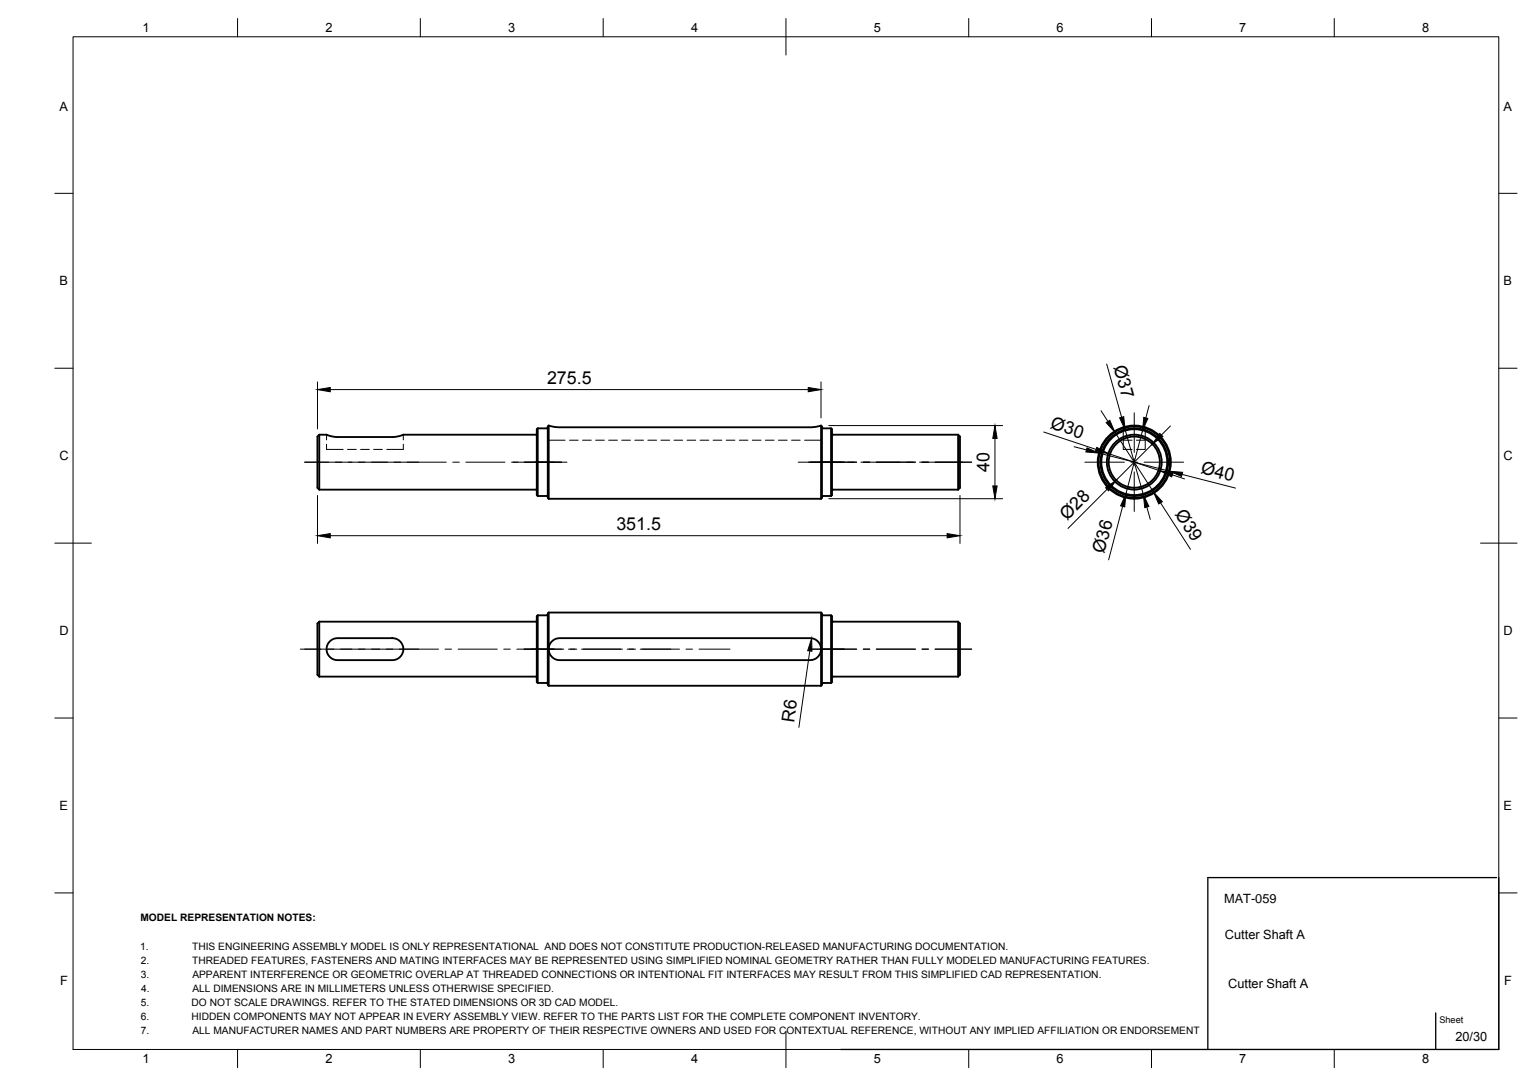
ISO-10303-21;
HEADER;
/* Generated by software containing ST-Developer
 * from STEP Tools, Inc. (www.steptools.com) 
 */

FILE_DESCRIPTION(
/* description */ ('', 'CAx-IF Rec.Pracs.---Representation and Presentation of Product Manufa
cturing Information (PMI)---4.0---2014-10-13'),
/* implementation_level */ '2;1');

FILE_NAME(
/* name */ 'Cutter Shaft A.step',
/* time_stamp */ '2026-10-28T23:00:48+01:00',
/* author */ (''),
/* organization */ (''),
/* preprocessor_version */ 'ST-DEVELOPER v20.2',
/* originating_system */ 'Autodesk Translation Framework v15.17.0.0',
/* authorisation */ '');

FILE_SCHEMA (('AP242_MANAGED_MODEL_BASED_3D_ENGINEERING_MIM_LF { 1 0 10303 442 2 1 4 }'));
ENDSEC;

DATA;
#10=MECHANICAL_DESIGN_GEOMETRIC_PRESENTATION_REPRESENTATION('',(#992),#61811);
#603=CONICAL_SURFACE('',#35992,18.25,0.785398163397426);
#604=CONICAL_SURFACE('',#35998,18.25,0.78539816339745);
#605=CONICAL_SURFACE('',#36004,14.5,0.785398163397442);
#606=CONICAL_SURFACE('',#36017,14.5,0.785398163397442);
#607=CONICAL_SURFACE('',#36025,19.75,0.78539816339745);
#608=CONICAL_SURFACE('',#36026,19.75,0.78539816339745);
#819=B_SPLINE_CURVE_WITH_KNOTS('',3,(#55896,#55897,#55898,#55899,#55900,
#55901,#55902,#55903,#55904,#55905),.UNSPECIFIED.,.F.,.F.,(4,2,2,2,4),(0.910129823137503,
1.1376283823127,1.36512694148791,1.59269329388146,1.82025964627501),
 .UNSPECIFIED.);
#820=B_SPLINE_CURVE_WITH_KNOTS('',3,(#55909,#55910,#55911,#55912,#55913,
#55914,#55915,#55916,#55917,#55918),.UNSPECIFIED.,.F.,.F.,(4,2,2,2,4),(1.82025964627501,
2.04782599866856,2.27539235106211,2.50289091023731,2.73038946941251),
 .UNSPECIFIED.);
#821=B_SPLINE_CURVE_WITH_KNOTS('',3,(#55923,#55924,#55925,#55926,#55927,
#55928,#55929,#55930,#55931,#55932,#55933,#55934,#55935,#55936,#55937,#55938,
#55939,#55940),.UNSPECIFIED.,.F.,.F.,(4,2,2,2,2,2,2,2,4),(0.,0.22893459915159,
0.45786919830318,0.68657220048275,0.91527520266232,1.14397820484189,1.37268120702146,
1.60161580617305,1.83055040532464),.UNSPECIFIED.);
#822=B_SPLINE_CURVE_WITH_KNOTS('',3,(#55959,#55960,#55961,#55962,#55963,
#55964,#55965,#55966,#55967,#55968,#55969,#55970,#55971,#55972,#55973,#55974,
#55975,#55976),.UNSPECIFIED.,.F.,.F.,(4,2,2,2,2,2,2,2,4),(-3.6611008106493,
-3.4321662114977,-3.20323161234611,-2.97452861016654,-2.74582560798697,
-2.5171226058074,-2.28841960362783,-2.05948500447624,-1.83055040532465),
 .UNSPECIFIED.);
#823=B_SPLINE_CURVE_WITH_KNOTS('',3,(#56047,#56048,#56049,#56050,#56051,
#56052,#56053,#56054,#56055,#56056),.UNSPECIFIED.,.F.,.F.,(4,2,2,2,4),(2.73038946941251,
2.95788802858771,3.18538658776291,3.41295294015646,3.64051929255001),
 .UNSPECIFIED.);
#824=B_SPLINE_CURVE_WITH_KNOTS('',3,(#56068,#56069,#56070,#56071,#56072,
#56073,#56074,#56075,#56076,#56077),.UNSPECIFIED.,.F.,.F.,(4,2,2,2,4),(0.,
0.22756635239355,0.4551327047871,0.682631263962301,0.910129823137503),
 .UNSPECIFIED.);
#898=TOROIDAL_SURFACE('',#35973,15.5,0.5);
#899=TOROIDAL_SURFACE('',#35982,15.5,0.5);
#900=TOROIDAL_SURFACE('',#36020,19.,0.500000000000029);
#901=TOROIDAL_SURFACE('',#36030,19.,0.499999999999998);
#928=SHAPE_REPRESENTATION_RELATIONSHIP('SRR','None',#61988,#953);
#953=ADVANCED_BREP_SHAPE_REPRESENTATION('',(#1031),#61801);
#992=STYLED_ITEM('',(#62156),#1031);
#1031=MANIFOLD_SOLID_BREP('Body1',#33822);
#1370=CYLINDRICAL_SURFACE('',#35963,20.);
#1371=CYLINDRICAL_SURFACE('',#35966,5.99999999999999);
#1372=CYLINDRICAL_SURFACE('',#35970,6.00000000000001);
#1373=CYLINDRICAL_SURFACE('',#35980,15.);
#1374=CYLINDRICAL_SURFACE('',#35989,15.);
#1375=CYLINDRICAL_SURFACE('',#35995,18.5);
#1376=CYLINDRICAL_SURFACE('',#36001,18.5);
#1377=CYLINDRICAL_SURFACE('',#36007,6.);
#1378=CYLINDRICAL_SURFACE('',#36011,6.);
#1379=CYLINDRICAL_SURFACE('',#36014,20.);
#2116=FACE_BOUND('',#7318,.T.);
#2117=FACE_BOUND('',#7320,.T.);
#2118=FACE_BOUND('',#7323,.T.);
#2119=FACE_BOUND('',#7341,.T.);
#2120=FACE_BOUND('',#7345,.T.);
#3038=CIRCLE('',#35964,20.);
#3039=CIRCLE('',#35965,20.);
#3040=CIRCLE('',#35967,5.99999999999999);
#3041=CIRCLE('',#35971,6.00000000000001);
#3042=CIRCLE('',#35974,15.);
#3043=CIRCLE('',#35975,15.);
#3044=CIRCLE('',#35976,0.5);
#3045=CIRCLE('',#35977,15.5);
#3046=CIRCLE('',#35979,18.);
#3047=CIRCLE('',#35981,15.);
#3048=CIRCLE('',#35983,15.5);
#3049=CIRCLE('',#35984,0.5);
#3050=CIRCLE('',#35985,15.);
#3051=CIRCLE('',#35986,15.);
#3052=CIRCLE('',#35988,18.);
#3053=CIRCLE('',#35990,15.);
#3054=CIRCLE('',#35991,15.);
#3055=CIRCLE('',#35993,18.5);
#3056=CIRCLE('',#35994,18.5);
#3057=CIRCLE('',#35996,18.5);
#3058=CIRCLE('',#35997,18.5);
#3059=CIRCLE('',#35999,18.5);
#3060=CIRCLE('',#36000,18.5);
#3061=CIRCLE('',#36002,18.5);
#3062=CIRCLE('',#36003,18.5);
#3063=CIRCLE('',#36005,14.);
#3064=CIRCLE('',#36008,6.);
#3065=CIRCLE('',#36012,6.);
#3066=CIRCLE('',#36015,20.);
#3067=CIRCLE('',#36016,20.);
#3068=CIRCLE('',#36018,14.);
#3069=CIRCLE('',#36021,19.);
#3070=CIRCLE('',#36022,0.500000000000029);
#3071=CIRCLE('',#36024,19.5);
#3072=CIRCLE('',#36027,19.5);
#3073=CIRCLE('',#36029,19.);
#3074=CIRCLE('',#36031,0.499999999999998);
#5194=FACE_OUTER_BOUND('',#7310,.T.);
#5195=FACE_OUTER_BOUND('',#7311,.T.);
#5196=FACE_OUTER_BOUND('',#7312,.T.);
#5197=FACE_OUTER_BOUND('',#7313,.T.);
#5198=FACE_OUTER_BOUND('',#7314,.T.);
#5199=FACE_OUTER_BOUND('',#7315,.T.);
#5200=FACE_OUTER_BOUND('',#7316,.T.);
#5201=FACE_OUTER_BOUND('',#7317,.T.);
#5202=FACE_OUTER_BOUND('',#7319,.T.);
#5203=FACE_OUTER_BOUND('',#7321,.T.);
#5204=FACE_OUTER_BOUND('',#7322,.T.);
#5205=FACE_OUTER_BOUND('',#7324,.T.);
#5206=FACE_OUTER_BOUND('',#7325,.T.);
#5207=FACE_OUTER_BOUND('',#7326,.T.);
#5208=FACE_OUTER_BOUND('',#7327,.T.);
#5209=FACE_OUTER_BOUND('',#7328,.T.);
#5210=FACE_OUTER_BOUND('',#7329,.T.);
#5211=FACE_OUTER_BOUND('',#7330,.T.);
#5212=FACE_OUTER_BOUND('',#7331,.T.);
#5213=FACE_OUTER_BOUND('',#7332,.T.);
#5214=FACE_OUTER_BOUND('',#7333,.T.);
#5215=FACE_OUTER_BOUND('',#7334,.T.);
#5216=FACE_OUTER_BOUND('',#7335,.T.);
#5217=FACE_OUTER_BOUND('',#7336,.T.);
#5218=FACE_OUTER_BOUND('',#7337,.T.);
#5219=FACE_OUTER_BOUND('',#7338,.T.);
#5220=FACE_OUTER_BOUND('',#7339,.T.);
#5221=FACE_OUTER_BOUND('',#7340,.T.);
#5222=FACE_OUTER_BOUND('',#7342,.T.);
#5223=FACE_OUTER_BOUND('',#7343,.T.);
#5224=FACE_OUTER_BOUND('',#7344,.T.);
#5225=FACE_OUTER_BOUND('',#7346,.T.);
#7310=EDGE_LOOP('',(#26242,#26243,#26244,#26245,#26246,#26247));
#7311=EDGE_LOOP('',(#26248,#26249,#26250,#26251));
#7312=EDGE_LOOP('',(#26252,#26253,#26254,#26255));
#7313=EDGE_LOOP('',(#26256,#26257,#26258,#26259));
#7314=EDGE_LOOP('',(#26260,#26261,#26262,#26263));
#7315=EDGE_LOOP('',(#26264,#26265,#26266,#26267));
#7316=EDGE_LOOP('',(#26268,#26269,#26270,#26271,#26272));
#7317=EDGE_LOOP('',(#26273));
#7318=EDGE_LOOP('',(#26274));
#7319=EDGE_LOOP('',(#26275,#26276,#26277,#26278,#26279));
#7320=EDGE_LOOP('',(#26280,#26281,#26282,#26283));
#7321=EDGE_LOOP('',(#26284,#26285,#26286,#26287,#26288));
#7322=EDGE_LOOP('',(#26289));
#7323=EDGE_LOOP('',(#26290));
#7324=EDGE_LOOP('',(#26291,#26292,#26293,#26294,#26295,#26296));
#7325=EDGE_LOOP('',(#26297,#26298,#26299,#26300,#26301));
#7326=EDGE_LOOP('',(#26302,#26303,#26304,#26305,#26306,#26307));
#7327=EDGE_LOOP('',(#26308,#26309,#26310,#26311,#26312));
#7328=EDGE_LOOP('',(#26313,#26314,#26315,#26316,#26317,#26318));
#7329=EDGE_LOOP('',(#26319,#26320,#26321,#26322,#26323));
#7330=EDGE_LOOP('',(#26324));
#7331=EDGE_LOOP('',(#26325,#26326,#26327,#26328,#26329));
#7332=EDGE_LOOP('',(#26330,#26331,#26332,#26333));
#7333=EDGE_LOOP('',(#26334,#26335,#26336,#26337));
#7334=EDGE_LOOP('',(#26338,#26339,#26340,#26341,#26342));
#7335=EDGE_LOOP('',(#26343,#26344,#26345,#26346));
#7336=EDGE_LOOP('',(#26347,#26348,#26349,#26350,#26351,#26352));
#7337=EDGE_LOOP('',(#26353,#26354,#26355,#26356));
#7338=EDGE_LOOP('',(#26357));
#7339=EDGE_LOOP('',(#26358,#26359,#26360,#26361,#26362));
#7340=EDGE_LOOP('',(#26363));
#7341=EDGE_LOOP('',(#26364));
#7342=EDGE_LOOP('',(#26365,#26366,#26367,#26368,#26369));
#7343=EDGE_LOOP('',(#26370,#26371,#26372,#26373,#26374));
#7344=EDGE_LOOP('',(#26375));
#7345=EDGE_LOOP('',(#26376));
#7346=EDGE_LOOP('',(#26377,#26378,#26379,#26380,#26381));
#9757=LINE('',#55892,#12304);
#9758=LINE('',#55907,#12305);
#9759=LINE('',#55942,#12306);
#9760=LINE('',#55945,#12307);
#9761=LINE('',#55948,#12308);
#9762=LINE('',#55950,#12309);
#9763=LINE('',#55951,#12310);
#9764=LINE('',#55954,#12311);
#9765=LINE('',#55956,#12312);
#9766=LINE('',#55957,#12313);
#9767=LINE('',#55993,#12314);
#9768=LINE('',#56007,#12315);
#9769=LINE('',#56016,#12316);
#9770=LINE('',#56021,#12317);
#9771=LINE('',#56028,#12318);
#9772=LINE('',#56031,#12319);
#9773=LINE('',#56037,#12320);
#9774=LINE('',#56042,#12321);
#9775=LINE('',#56046,#12322);
#9776=LINE('',#56059,#12323);
#9777=LINE('',#56061,#12324);
#9778=LINE('',#56062,#12325);
#9779=LINE('',#56065,#12326);
#9780=LINE('',#56066,#12327);
#9781=LINE('',#56085,#12328);
#9782=LINE('',#56096,#12329);
#9783=LINE('',#56099,#12330);
#12304=VECTOR('',#43281,20.);
#12305=VECTOR('',#43284,10.);
#12306=VECTOR('',#43289,10.);
#12307=VECTOR('',#43292,10.);
#12308=VECTOR('',#43295,10.);
#12309=VECTOR('',#43296,10.);
#12310=VECTOR('',#43297,10.);
#12311=VECTOR('',#43300,10.);
#12312=VECTOR('',#43301,10.);
#12313=VECTOR('',#43302,10.);
#12314=VECTOR('',#43327,15.);
#12315=VECTOR('',#43344,15.);
#12316=VECTOR('',#43355,18.25);
#12317=VECTOR('',#43360,18.5);
#12318=VECTOR('',#43369,18.25);
#12319=VECTOR('',#43372,18.5);
#12320=VECTOR('',#43379,14.5);
#12321=VECTOR('',#43386,10.);
#12322=VECTOR('',#43389,10.);
#12323=VECTOR('',#43392,10.);
#12324=VECTOR('',#43393,10.);
#12325=VECTOR('',#43394,10.);
#12326=VECTOR('',#43397,10.);
#12327=VECTOR('',#43398,10.);
#12328=VECTOR('',#43413,14.5);
#12329=VECTOR('',#43430,19.75);
#12330=VECTOR('',#43433,19.75);
#15002=VERTEX_POINT('',#55890);
#15003=VERTEX_POINT('',#55891);
#15004=VERTEX_POINT('',#55893);
#15005=VERTEX_POINT('',#55895);
#15006=VERTEX_POINT('',#55906);
#15007=VERTEX_POINT('',#55908);
#15008=VERTEX_POINT('',#55921);
#15009=VERTEX_POINT('',#55922);
#15010=VERTEX_POINT('',#55941);
#15011=VERTEX_POINT('',#55943);
#15012=VERTEX_POINT('',#55947);
#15013=VERTEX_POINT('',#55949);
#15014=VERTEX_POINT('',#55953);
#15015=VERTEX_POINT('',#55955);
#15016=VERTEX_POINT('',#55980);
#15017=VERTEX_POINT('',#55981);
#15018=VERTEX_POINT('',#55984);
#15019=VERTEX_POINT('',#55988);
#15020=VERTEX_POINT('',#55991);
#15021=VERTEX_POINT('',#55995);
#15022=VERTEX_POINT('',#55997);
#15023=VERTEX_POINT('',#55999);
#15024=VERTEX_POINT('',#56003);
#15025=VERTEX_POINT('',#56006);
#15026=VERTEX_POINT('',#56008);
#15027=VERTEX_POINT('',#56012);
#15028=VERTEX_POINT('',#56013);
#15029=VERTEX_POINT('',#56018);
#15030=VERTEX_POINT('',#56019);
#15031=VERTEX_POINT('',#56024);
#15032=VERTEX_POINT('',#56025);
#15033=VERTEX_POINT('',#56030);
#15034=VERTEX_POINT('',#56032);
#15035=VERTEX_POINT('',#56036);
#15036=VERTEX_POINT('',#56041);
#15037=VERTEX_POINT('',#56043);
#15038=VERTEX_POINT('',#56045);
#15039=VERTEX_POINT('',#56058);
#15040=VERTEX_POINT('',#56060);
#15041=VERTEX_POINT('',#56064);
#15042=VERTEX_POINT('',#56084);
#15043=VERTEX_POINT('',#56089);
#15044=VERTEX_POINT('',#56093);
#15045=VERTEX_POINT('',#56098);
#15046=VERTEX_POINT('',#56102);
#19023=EDGE_CURVE('',#15002,#15003,#9757,.T.);
#19024=EDGE_CURVE('',#15004,#15002,#3038,.T.);
#19025=EDGE_CURVE('',#15004,#15005,#819,.T.);
#19026=EDGE_CURVE('',#15005,#15006,#9758,.T.);
#19027=EDGE_CURVE('',#15006,#15007,#820,.T.);
#19028=EDGE_CURVE('',#15007,#15003,#3039,.T.);
#19029=EDGE_CURVE('',#15008,#15009,#821,.T.);
#19030=EDGE_CURVE('',#15008,#15010,#9759,.T.);
#19031=EDGE_CURVE('',#15010,#15011,#3040,.T.);
#19032=EDGE_CURVE('',#15009,#15011,#9760,.T.);
#19033=EDGE_CURVE('',#15009,#15012,#9761,.T.);
#19034=EDGE_CURVE('',#15011,#15013,#9762,.T.);
#19035=EDGE_CURVE('',#15012,#15013,#9763,.T.);
#19036=EDGE_CURVE('',#15014,#15008,#9764,.T.);
#19037=EDGE_CURVE('',#15014,#15015,#9765,.T.);
#19038=EDGE_CURVE('',#15015,#15010,#9766,.T.);
#19039=EDGE_CURVE('',#15012,#15014,#822,.F.);
#19040=EDGE_CURVE('',#15013,#15015,#3041,.T.);
#19041=EDGE_CURVE('',#15016,#15017,#3042,.T.);
#19042=EDGE_CURVE('',#15017,#15016,#3043,.T.);
#19043=EDGE_CURVE('',#15016,#15018,#3044,.T.);
#19044=EDGE_CURVE('',#15018,#15018,#3045,.T.);
#19045=EDGE_CURVE('',#15019,#15019,#3046,.T.);
#19046=EDGE_CURVE('',#15020,#15020,#3047,.T.);
#19047=EDGE_CURVE('',#15020,#15017,#9767,.T.);
#19048=EDGE_CURVE('',#15021,#15021,#3048,.T.);
#19049=EDGE_CURVE('',#15021,#15022,#3049,.T.);
#19050=EDGE_CURVE('',#15022,#15023,#3050,.T.);
#19051=EDGE_CURVE('',#15023,#15022,#3051,.T.);
#19052=EDGE_CURVE('',#15024,#15024,#3052,.T.);
#19053=EDGE_CURVE('',#15023,#15025,#9768,.T.);
#19054=EDGE_CURVE('',#15026,#15025,#3053,.T.);
#19055=EDGE_CURVE('',#15025,#15026,#3054,.T.);
#19056=EDGE_CURVE('',#15027,#15028,#3055,.T.);
#19057=EDGE_CURVE('',#15028,#15027,#3056,.T.);
#19058=EDGE_CURVE('',#15027,#15024,#9769,.T.);
#19059=EDGE_CURVE('',#15029,#15030,#3057,.T.);
#19060=EDGE_CURVE('',#15029,#15028,#9770,.T.);
#19061=EDGE_CURVE('',#15030,#15029,#3058,.T.);
#19062=EDGE_CURVE('',#15031,#15032,#3059,.T.);
#19063=EDGE_CURVE('',#15032,#15031,#3060,.T.);
#19064=EDGE_CURVE('',#15031,#15019,#9771,.T.);
#19065=EDGE_CURVE('',#15032,#15033,#9772,.T.);
#19066=EDGE_CURVE('',#15033,#15034,#3061,.T.);
#19067=EDGE_CURVE('',#15034,#15033,#3062,.T.);
#19068=EDGE_CURVE('',#15026,#15035,#9773,.T.);
#19069=EDGE_CURVE('',#15035,#15035,#3063,.T.);
#19070=EDGE_CURVE('',#15006,#15036,#9774,.T.);
#19071=EDGE_CURVE('',#15036,#15037,#3064,.T.);
#19072=EDGE_CURVE('',#15038,#15037,#9775,.T.);
#19073=EDGE_CURVE('',#15007,#15038,#823,.T.);
#19074=EDGE_CURVE('',#15038,#15039,#9776,.T.);
#19075=EDGE_CURVE('',#15037,#15040,#9777,.T.);
#19076=EDGE_CURVE('',#15039,#15040,#9778,.T.);
#19077=EDGE_CURVE('',#15005,#15041,#9779,.T.);
#19078=EDGE_CURVE('',#15041,#15036,#9780,.T.);
#19079=EDGE_CURVE('',#15039,#15004,#824,.T.);
#19080=EDGE_CURVE('',#15040,#15041,#3065,.T.);
#19081=EDGE_CURVE('',#15003,#15007,#3066,.T.);
#19082=EDGE_CURVE('',#15002,#15004,#3067,.T.);
#19083=EDGE_CURVE('',#15020,#15042,#9781,.T.);
#19084=EDGE_CURVE('',#15042,#15042,#3068,.T.);
#19085=EDGE_CURVE('',#15043,#15043,#3069,.T.);
#19086=EDGE_CURVE('',#15043,#15030,#3070,.T.);
#19087=EDGE_CURVE('',#15044,#15044,#3071,.T.);
#19088=EDGE_CURVE('',#15003,#15044,#9782,.T.);
#19089=EDGE_CURVE('',#15002,#15045,#9783,.T.);
#19090=EDGE_CURVE('',#15045,#15045,#3072,.T.);
#19091=EDGE_CURVE('',#15046,#15046,#3073,.T.);
#19092=EDGE_CURVE('',#15034,#15046,#3074,.T.);
#26242=ORIENTED_EDGE('',*,*,#19023,.F.);
#26243=ORIENTED_EDGE('',*,*,#19024,.F.);
#26244=ORIENTED_EDGE('',*,*,#19025,.T.);
#26245=ORIENTED_EDGE('',*,*,#19026,.T.);
#26246=ORIENTED_EDGE('',*,*,#19027,.T.);
#26247=ORIENTED_EDGE('',*,*,#19028,.T.);
#26248=ORIENTED_EDGE('',*,*,#19029,.F.);
#26249=ORIENTED_EDGE('',*,*,#19030,.T.);
#26250=ORIENTED_EDGE('',*,*,#19031,.T.);
#26251=ORIENTED_EDGE('',*,*,#19032,.F.);
#26252=ORIENTED_EDGE('',*,*,#19033,.F.);
#26253=ORIENTED_EDGE('',*,*,#19032,.T.);
#26254=ORIENTED_EDGE('',*,*,#19034,.T.);
#26255=ORIENTED_EDGE('',*,*,#19035,.F.);
#26256=ORIENTED_EDGE('',*,*,#19036,.F.);
#26257=ORIENTED_EDGE('',*,*,#19037,.T.);
#26258=ORIENTED_EDGE('',*,*,#19038,.T.);
#26259=ORIENTED_EDGE('',*,*,#19030,.F.);
#26260=ORIENTED_EDGE('',*,*,#19039,.F.);
#26261=ORIENTED_EDGE('',*,*,#19035,.T.);
#26262=ORIENTED_EDGE('',*,*,#19040,.T.);
#26263=ORIENTED_EDGE('',*,*,#19037,.F.);
#26264=ORIENTED_EDGE('',*,*,#19034,.F.);
#26265=ORIENTED_EDGE('',*,*,#19031,.F.);
#26266=ORIENTED_EDGE('',*,*,#19038,.F.);
#26267=ORIENTED_EDGE('',*,*,#19040,.F.);
#26268=ORIENTED_EDGE('',*,*,#19041,.T.);
#26269=ORIENTED_EDGE('',*,*,#19042,.T.);
#26270=ORIENTED_EDGE('',*,*,#19043,.T.);
#26271=ORIENTED_EDGE('',*,*,#19044,.T.);
#26272=ORIENTED_EDGE('',*,*,#19043,.F.);
#26273=ORIENTED_EDGE('',*,*,#19045,.F.);
#26274=ORIENTED_EDGE('',*,*,#19044,.F.);
#26275=ORIENTED_EDGE('',*,*,#19046,.F.);
#26276=ORIENTED_EDGE('',*,*,#19047,.T.);
#26277=ORIENTED_EDGE('',*,*,#19041,.F.);
#26278=ORIENTED_EDGE('',*,*,#19042,.F.);
#26279=ORIENTED_EDGE('',*,*,#19047,.F.);
#26280=ORIENTED_EDGE('',*,*,#19039,.T.);
#26281=ORIENTED_EDGE('',*,*,#19036,.T.);
#26282=ORIENTED_EDGE('',*,*,#19029,.T.);
#26283=ORIENTED_EDGE('',*,*,#19033,.T.);
#26284=ORIENTED_EDGE('',*,*,#19048,.T.);
#26285=ORIENTED_EDGE('',*,*,#19049,.T.);
#26286=ORIENTED_EDGE('',*,*,#19050,.T.);
#26287=ORIENTED_EDGE('',*,*,#19051,.T.);
#26288=ORIENTED_EDGE('',*,*,#19049,.F.);
#26289=ORIENTED_EDGE('',*,*,#19052,.F.);
#26290=ORIENTED_EDGE('',*,*,#19048,.F.);
#26291=ORIENTED_EDGE('',*,*,#19051,.F.);
#26292=ORIENTED_EDGE('',*,*,#19053,.T.);
#26293=ORIENTED_EDGE('',*,*,#19054,.F.);
#26294=ORIENTED_EDGE('',*,*,#19055,.F.);
#26295=ORIENTED_EDGE('',*,*,#19053,.F.);
#26296=ORIENTED_EDGE('',*,*,#19050,.F.);
#26297=ORIENTED_EDGE('',*,*,#19056,.T.);
#26298=ORIENTED_EDGE('',*,*,#19057,.T.);
#26299=ORIENTED_EDGE('',*,*,#19058,.T.);
#26300=ORIENTED_EDGE('',*,*,#19052,.T.);
#26301=ORIENTED_EDGE('',*,*,#19058,.F.);
#26302=ORIENTED_EDGE('',*,*,#19059,.F.);
#26303=ORIENTED_EDGE('',*,*,#19060,.T.);
#26304=ORIENTED_EDGE('',*,*,#19056,.F.);
#26305=ORIENTED_EDGE('',*,*,#19057,.F.);
#26306=ORIENTED_EDGE('',*,*,#19060,.F.);
#26307=ORIENTED_EDGE('',*,*,#19061,.F.);
#26308=ORIENTED_EDGE('',*,*,#19062,.T.);
#26309=ORIENTED_EDGE('',*,*,#19063,.T.);
#26310=ORIENTED_EDGE('',*,*,#19064,.T.);
#26311=ORIENTED_EDGE('',*,*,#19045,.T.);
#26312=ORIENTED_EDGE('',*,*,#19064,.F.);
#26313=ORIENTED_EDGE('',*,*,#19062,.F.);
#26314=ORIENTED_EDGE('',*,*,#19063,.F.);
#26315=ORIENTED_EDGE('',*,*,#19065,.T.);
#26316=ORIENTED_EDGE('',*,*,#19066,.T.);
#26317=ORIENTED_EDGE('',*,*,#19067,.T.);
#26318=ORIENTED_EDGE('',*,*,#19065,.F.);
#26319=ORIENTED_EDGE('',*,*,#19054,.T.);
#26320=ORIENTED_EDGE('',*,*,#19055,.T.);
#26321=ORIENTED_EDGE('',*,*,#19068,.T.);
#26322=ORIENTED_EDGE('',*,*,#19069,.T.);
#26323=ORIENTED_EDGE('',*,*,#19068,.F.);
#26324=ORIENTED_EDGE('',*,*,#19069,.F.);
#26325=ORIENTED_EDGE('',*,*,#19027,.F.);
#26326=ORIENTED_EDGE('',*,*,#19070,.T.);
#26327=ORIENTED_EDGE('',*,*,#19071,.T.);
#26328=ORIENTED_EDGE('',*,*,#19072,.F.);
#26329=ORIENTED_EDGE('',*,*,#19073,.F.);
#26330=ORIENTED_EDGE('',*,*,#19074,.F.);
#26331=ORIENTED_EDGE('',*,*,#19072,.T.);
#26332=ORIENTED_EDGE('',*,*,#19075,.T.);
#26333=ORIENTED_EDGE('',*,*,#19076,.F.);
#26334=ORIENTED_EDGE('',*,*,#19026,.F.);
#26335=ORIENTED_EDGE('',*,*,#19077,.T.);
#26336=ORIENTED_EDGE('',*,*,#19078,.T.);
#26337=ORIENTED_EDGE('',*,*,#19070,.F.);
#26338=ORIENTED_EDGE('',*,*,#19025,.F.);
#26339=ORIENTED_EDGE('',*,*,#19079,.F.);
#26340=ORIENTED_EDGE('',*,*,#19076,.T.);
#26341=ORIENTED_EDGE('',*,*,#19080,.T.);
#26342=ORIENTED_EDGE('',*,*,#19077,.F.);
#26343=ORIENTED_EDGE('',*,*,#19071,.F.);
#26344=ORIENTED_EDGE('',*,*,#19078,.F.);
#26345=ORIENTED_EDGE('',*,*,#19080,.F.);
#26346=ORIENTED_EDGE('',*,*,#19075,.F.);
#26347=ORIENTED_EDGE('',*,*,#19023,.T.);
#26348=ORIENTED_EDGE('',*,*,#19081,.T.);
#26349=ORIENTED_EDGE('',*,*,#19073,.T.);
#26350=ORIENTED_EDGE('',*,*,#19074,.T.);
#26351=ORIENTED_EDGE('',*,*,#19079,.T.);
#26352=ORIENTED_EDGE('',*,*,#19082,.F.);
#26353=ORIENTED_EDGE('',*,*,#19046,.T.);
#26354=ORIENTED_EDGE('',*,*,#19083,.T.);
#26355=ORIENTED_EDGE('',*,*,#19084,.F.);
#26356=ORIENTED_EDGE('',*,*,#19083,.F.);
#26357=ORIENTED_EDGE('',*,*,#19084,.T.);
#26358=ORIENTED_EDGE('',*,*,#19085,.F.);
#26359=ORIENTED_EDGE('',*,*,#19086,.T.);
#26360=ORIENTED_EDGE('',*,*,#19061,.T.);
#26361=ORIENTED_EDGE('',*,*,#19059,.T.);
#26362=ORIENTED_EDGE('',*,*,#19086,.F.);
#26363=ORIENTED_EDGE('',*,*,#19087,.F.);
#26364=ORIENTED_EDGE('',*,*,#19085,.T.);
#26365=ORIENTED_EDGE('',*,*,#19028,.F.);
#26366=ORIENTED_EDGE('',*,*,#19081,.F.);
#26367=ORIENTED_EDGE('',*,*,#19088,.T.);
#26368=ORIENTED_EDGE('',*,*,#19087,.T.);
#26369=ORIENTED_EDGE('',*,*,#19088,.F.);
#26370=ORIENTED_EDGE('',*,*,#19024,.T.);
#26371=ORIENTED_EDGE('',*,*,#19089,.T.);
#26372=ORIENTED_EDGE('',*,*,#19090,.F.);
#26373=ORIENTED_EDGE('',*,*,#19089,.F.);
#26374=ORIENTED_EDGE('',*,*,#19082,.T.);
#26375=ORIENTED_EDGE('',*,*,#19090,.T.);
#26376=ORIENTED_EDGE('',*,*,#19091,.F.);
#26377=ORIENTED_EDGE('',*,*,#19066,.F.);
#26378=ORIENTED_EDGE('',*,*,#19067,.F.);
#26379=ORIENTED_EDGE('',*,*,#19092,.T.);
#26380=ORIENTED_EDGE('',*,*,#19091,.T.);
#26381=ORIENTED_EDGE('',*,*,#19092,.F.);
#31625=PLANE('',#35968);
#31626=PLANE('',#35969);
#31627=PLANE('',#35972);
#31628=PLANE('',#35978);
#31629=PLANE('',#35987);
#31630=PLANE('',#36006);
#31631=PLANE('',#36009);
#31632=PLANE('',#36010);
#31633=PLANE('',#36013);
#31634=PLANE('',#36019);
#31635=PLANE('',#36023);
#31636=PLANE('',#36028);
#32875=ADVANCED_FACE('',(#5194),#1370,.T.);
#32876=ADVANCED_FACE('',(#5195),#1371,.F.);
#32877=ADVANCED_FACE('',(#5196),#31625,.F.);
#32878=ADVANCED_FACE('',(#5197),#31626,.F.);
#32879=ADVANCED_FACE('',(#5198),#1372,.F.);
#32880=ADVANCED_FACE('',(#5199),#31627,.F.);
#32881=ADVANCED_FACE('',(#5200),#898,.F.);
#32882=ADVANCED_FACE('',(#5201,#2116),#31628,.T.);
#32883=ADVANCED_FACE('',(#5202,#2117),#1373,.T.);
#32884=ADVANCED_FACE('',(#5203),#899,.F.);
#32885=ADVANCED_FACE('',(#5204,#2118),#31629,.T.);
#32886=ADVANCED_FACE('',(#5205),#1374,.T.);
#32887=ADVANCED_FACE('',(#5206),#603,.T.);
#32888=ADVANCED_FACE('',(#5207),#1375,.T.);
#32889=ADVANCED_FACE('',(#5208),#604,.T.);
#32890=ADVANCED_FACE('',(#5209),#1376,.T.);
#32891=ADVANCED_FACE('',(#5210),#605,.T.);
#32892=ADVANCED_FACE('',(#5211),#31630,.T.);
#32893=ADVANCED_FACE('',(#5212),#1377,.F.);
#32894=ADVANCED_FACE('',(#5213),#31631,.F.);
#32895=ADVANCED_FACE('',(#5214),#31632,.F.);
#32896=ADVANCED_FACE('',(#5215),#1378,.F.);
#32897=ADVANCED_FACE('',(#5216),#31633,.T.);
#32898=ADVANCED_FACE('',(#5217),#1379,.T.);
#32899=ADVANCED_FACE('',(#5218),#606,.T.);
#32900=ADVANCED_FACE('',(#5219),#31634,.T.);
#32901=ADVANCED_FACE('',(#5220),#900,.F.);
#32902=ADVANCED_FACE('',(#5221,#2119),#31635,.T.);
#32903=ADVANCED_FACE('',(#5222),#607,.T.);
#32904=ADVANCED_FACE('',(#5223),#608,.T.);
#32905=ADVANCED_FACE('',(#5224,#2120),#31636,.T.);
#32906=ADVANCED_FACE('',(#5225),#901,.F.);
#33822=CLOSED_SHELL('',(#32875,#32876,#32877,#32878,#32879,#32880,#32881,
#32882,#32883,#32884,#32885,#32886,#32887,#32888,#32889,#32890,#32891,#32892,
#32893,#32894,#32895,#32896,#32897,#32898,#32899,#32900,#32901,#32902,#32903,
#32904,#32905,#32906));
#35962=AXIS2_PLACEMENT_3D('',#55888,#43277,#43278);
#35963=AXIS2_PLACEMENT_3D('',#55889,#43279,#43280);
#35964=AXIS2_PLACEMENT_3D('',#55894,#43282,#43283);
#35965=AXIS2_PLACEMENT_3D('',#55919,#43285,#43286);
#35966=AXIS2_PLACEMENT_3D('',#55920,#43287,#43288);
#35967=AXIS2_PLACEMENT_3D('',#55944,#43290,#43291);
#35968=AXIS2_PLACEMENT_3D('',#55946,#43293,#43294);
#35969=AXIS2_PLACEMENT_3D('',#55952,#43298,#43299);
#35970=AXIS2_PLACEMENT_3D('',#55958,#43303,#43304);
#35971=AXIS2_PLACEMENT_3D('',#55977,#43305,#43306);
#35972=AXIS2_PLACEMENT_3D('',#55978,#43307,#43308);
#35973=AXIS2_PLACEMENT_3D('',#55979,#43309,#43310);
#35974=AXIS2_PLACEMENT_3D('',#55982,#43311,#43312);
#35975=AXIS2_PLACEMENT_3D('',#55983,#43313,#43314);
#35976=AXIS2_PLACEMENT_3D('',#55985,#43315,#43316);
#35977=AXIS2_PLACEMENT_3D('',#55986,#43317,#43318);
#35978=AXIS2_PLACEMENT_3D('',#55987,#43319,#43320);
#35979=AXIS2_PLACEMENT_3D('',#55989,#43321,#43322);
#35980=AXIS2_PLACEMENT_3D('',#55990,#43323,#43324);
#35981=AXIS2_PLACEMENT_3D('',#55992,#43325,#43326);
#35982=AXIS2_PLACEMENT_3D('',#55994,#43328,#43329);
#35983=AXIS2_PLACEMENT_3D('',#55996,#43330,#43331);
#35984=AXIS2_PLACEMENT_3D('',#55998,#43332,#43333);
#35985=AXIS2_PLACEMENT_3D('',#56000,#43334,#43335);
#35986=AXIS2_PLACEMENT_3D('',#56001,#43336,#43337);
#35987=AXIS2_PLACEMENT_3D('',#56002,#43338,#43339);
#35988=AXIS2_PLACEMENT_3D('',#56004,#43340,#43341);
#35989=AXIS2_PLACEMENT_3D('',#56005,#43342,#43343);
#35990=AXIS2_PLACEMENT_3D('',#56009,#43345,#43346);
#35991=AXIS2_PLACEMENT_3D('',#56010,#43347,#43348);
#35992=AXIS2_PLACEMENT_3D('',#56011,#43349,#43350);
#35993=AXIS2_PLACEMENT_3D('',#56014,#43351,#43352);
#35994=AXIS2_PLACEMENT_3D('',#56015,#43353,#43354);
#35995=AXIS2_PLACEMENT_3D('',#56017,#43356,#43357);
#35996=AXIS2_PLACEMENT_3D('',#56020,#43358,#43359);
#35997=AXIS2_PLACEMENT_3D('',#56022,#43361,#43362);
#35998=AXIS2_PLACEMENT_3D('',#56023,#43363,#43364);
#35999=AXIS2_PLACEMENT_3D('',#56026,#43365,#43366);
#36000=AXIS2_PLACEMENT_3D('',#56027,#43367,#43368);
#36001=AXIS2_PLACEMENT_3D('',#56029,#43370,#43371);
#36002=AXIS2_PLACEMENT_3D('',#56033,#43373,#43374);
#36003=AXIS2_PLACEMENT_3D('',#56034,#43375,#43376);
#36004=AXIS2_PLACEMENT_3D('',#56035,#43377,#43378);
#36005=AXIS2_PLACEMENT_3D('',#56038,#43380,#43381);
#36006=AXIS2_PLACEMENT_3D('',#56039,#43382,#43383);
#36007=AXIS2_PLACEMENT_3D('',#56040,#43384,#43385);
#36008=AXIS2_PLACEMENT_3D('',#56044,#43387,#43388);
#36009=AXIS2_PLACEMENT_3D('',#56057,#43390,#43391);
#36010=AXIS2_PLACEMENT_3D('',#56063,#43395,#43396);
#36011=AXIS2_PLACEMENT_3D('',#56067,#43399,#43400);
#36012=AXIS2_PLACEMENT_3D('',#56078,#43401,#43402);
#36013=AXIS2_PLACEMENT_3D('',#56079,#43403,#43404);
#36014=AXIS2_PLACEMENT_3D('',#56080,#43405,#43406);
#36015=AXIS2_PLACEMENT_3D('',#56081,#43407,#43408);
#36016=AXIS2_PLACEMENT_3D('',#56082,#43409,#43410);
#36017=AXIS2_PLACEMENT_3D('',#56083,#43411,#43412);
#36018=AXIS2_PLACEMENT_3D('',#56086,#43414,#43415);
#36019=AXIS2_PLACEMENT_3D('',#56087,#43416,#43417);
#36020=AXIS2_PLACEMENT_3D('',#56088,#43418,#43419);
#36021=AXIS2_PLACEMENT_3D('',#56090,#43420,#43421);
#36022=AXIS2_PLACEMENT_3D('',#56091,#43422,#43423);
#36023=AXIS2_PLACEMENT_3D('',#56092,#43424,#43425);
#36024=AXIS2_PLACEMENT_3D('',#56094,#43426,#43427);
#36025=AXIS2_PLACEMENT_3D('',#56095,#43428,#43429);
#36026=AXIS2_PLACEMENT_3D('',#56097,#43431,#43432);
#36027=AXIS2_PLACEMENT_3D('',#56100,#43434,#43435);
#36028=AXIS2_PLACEMENT_3D('',#56101,#43436,#43437);
#36029=AXIS2_PLACEMENT_3D('',#56103,#43438,#43439);
#36030=AXIS2_PLACEMENT_3D('',#56104,#43440,#43441);
#36031=AXIS2_PLACEMENT_3D('',#56105,#43442,#43443);
#43277=DIRECTION('axis',(0.,0.,1.));
#43278=DIRECTION('refdir',(1.,0.,0.));
#43279=DIRECTION('center_axis',(4.88578146679885E-16,1.,-9.3381869947186E-16));
#43280=DIRECTION('ref_axis',(1.,-4.8857814667989E-16,-5.46077161851014E-15));
#43281=DIRECTION('',(-4.88578146679885E-16,-1.,9.3381869947186E-16));
#43282=DIRECTION('center_axis',(4.88578146679885E-16,1.,-9.3381869947186E-16));
#43283=DIRECTION('ref_axis',(5.46077161851014E-15,9.33818699471857E-16,
1.));
#43284=DIRECTION('',(-4.88578146679885E-16,-1.,9.3381869947186E-16));
#43285=DIRECTION('center_axis',(4.88578146679885E-16,1.,-9.3381869947186E-16));
#43286=DIRECTION('ref_axis',(5.46077161851014E-15,9.33818699471857E-16,
1.));
#43287=DIRECTION('center_axis',(-1.,4.8857814667989E-16,5.46077161851014E-15));
#43288=DIRECTION('ref_axis',(4.88578146679884E-16,1.,-1.0562833793866E-15));
#43289=DIRECTION('',(-1.,4.8857814667989E-16,5.46077161851014E-15));
#43290=DIRECTION('center_axis',(-1.,4.8857814667989E-16,5.46077161851014E-15));
#43291=DIRECTION('ref_axis',(-4.88578146679885E-16,-1.,9.3381869947186E-16));
#43292=DIRECTION('',(-1.,4.8857814667989E-16,5.46077161851014E-15));
#43293=DIRECTION('center_axis',(-5.46077161851014E-15,-1.34090047516775E-15,
-1.));
#43294=DIRECTION('ref_axis',(-4.88578146679883E-16,-1.,1.34090047516775E-15));
#43295=DIRECTION('',(-4.88578146679885E-16,-1.,9.3381869947186E-16));
#43296=DIRECTION('',(-4.88578146679883E-16,-1.,1.34090047516775E-15));
#43297=DIRECTION('',(-1.,4.8857814667989E-16,5.46077161851014E-15));
#43298=DIRECTION('center_axis',(5.46077161851014E-15,1.2668856068594E-15,
1.));
#43299=DIRECTION('ref_axis',(4.88578146679883E-16,1.,-1.26688560685941E-15));
#43300=DIRECTION('',(4.88578146679885E-16,1.,-9.3381869947186E-16));
#43301=DIRECTION('',(-1.,4.8857814667989E-16,5.46077161851014E-15));
#43302=DIRECTION('',(4.88578146679883E-16,1.,-1.26688560685941E-15));
#43303=DIRECTION('center_axis',(-1.,4.8857814667989E-16,5.46077161851014E-15));
#43304=DIRECTION('ref_axis',(-4.88578146679885E-16,-1.,9.3381869947186E-16));
#43305=DIRECTION('center_axis',(-1.,4.8857814667989E-16,5.46077161851014E-15));
#43306=DIRECTION('ref_axis',(-4.88578146679885E-16,-1.,9.3381869947186E-16));
#43307=DIRECTION('center_axis',(-1.,4.14563278371546E-16,5.46077161851014E-15));
#43308=DIRECTION('ref_axis',(5.46077161851014E-15,9.33818699471857E-16,
1.));
#43309=DIRECTION('center_axis',(4.88578146679885E-16,1.,-9.3381869947186E-16));
#43310=DIRECTION('ref_axis',(3.5527136788005E-15,8.88178419700125E-16,1.));
#43311=DIRECTION('center_axis',(-4.88578146679885E-16,-1.,9.3381869947186E-16));
#43312=DIRECTION('ref_axis',(-1.,4.8857814667989E-16,5.27707459863804E-15));
#43313=DIRECTION('center_axis',(-4.88578146679885E-16,-1.,9.3381869947186E-16));
#43314=DIRECTION('ref_axis',(-1.,4.8857814667989E-16,5.27707459863804E-15));
#43315=DIRECTION('center_axis',(1.,-4.88578146679891E-16,-6.66133814775093E-15));
#43316=DIRECTION('ref_axis',(-6.66133814775093E-15,-1.11022302462516E-15,
-1.));
#43317=DIRECTION('center_axis',(4.88578146679885E-16,1.,-9.3381869947186E-16));
#43318=DIRECTION('ref_axis',(-1.,4.8857814667989E-16,5.27707459863804E-15));
#43319=DIRECTION('center_axis',(4.88578146679885E-16,1.,-9.3381869947186E-16));
#43320=DIRECTION('ref_axis',(5.46077161851014E-15,9.33818699471857E-16,
1.));
#43321=DIRECTION('center_axis',(-4.88578146679885E-16,-1.,9.3381869947186E-16));
#43322=DIRECTION('ref_axis',(-1.,4.8857814667989E-16,5.46077161851014E-15));
#43323=DIRECTION('center_axis',(4.88578146679885E-16,1.,-9.3381869947186E-16));
#43324=DIRECTION('ref_axis',(1.,-4.8857814667989E-16,-5.46077161851014E-15));
#43325=DIRECTION('center_axis',(4.88578146679885E-16,1.,-9.3381869947186E-16));
#43326=DIRECTION('ref_axis',(5.46077161851014E-15,9.33818699471857E-16,
1.));
#43327=DIRECTION('',(-4.88578146679885E-16,-1.,9.3381869947186E-16));
#43328=DIRECTION('center_axis',(4.88578146679885E-16,1.,-9.3381869947186E-16));
#43329=DIRECTION('ref_axis',(3.5527136788005E-15,0.,1.));
#43330=DIRECTION('center_axis',(-4.88578146679885E-16,-1.,9.3381869947186E-16));
#43331=DIRECTION('ref_axis',(-1.,4.8857814667989E-16,5.27707459863804E-15));
#43332=DIRECTION('center_axis',(1.,-4.88578146679891E-16,-6.66133814775093E-15));
#43333=DIRECTION('ref_axis',(-6.66133814775093E-15,0.,-1.));
#43334=DIRECTION('center_axis',(4.88578146679885E-16,1.,-9.3381869947186E-16));
#43335=DIRECTION('ref_axis',(-1.,4.8857814667989E-16,5.27707459863804E-15));
#43336=DIRECTION('center_axis',(4.88578146679885E-16,1.,-9.3381869947186E-16));
#43337=DIRECTION('ref_axis',(-1.,4.8857814667989E-16,5.27707459863804E-15));
#43338=DIRECTION('center_axis',(-4.88578146679885E-16,-1.,9.3381869947186E-16));
#43339=DIRECTION('ref_axis',(-5.46077161851014E-15,-9.33818699471857E-16,
-1.));
#43340=DIRECTION('center_axis',(4.88578146679885E-16,1.,-9.3381869947186E-16));
#43341=DIRECTION('ref_axis',(-1.,4.8857814667989E-16,5.46077161851014E-15));
#43342=DIRECTION('center_axis',(4.88578146679885E-16,1.,-9.3381869947186E-16));
#43343=DIRECTION('ref_axis',(1.,-4.8857814667989E-16,-5.46077161851014E-15));
#43344=DIRECTION('',(-4.88578146679885E-16,-1.,9.3381869947186E-16));
#43345=DIRECTION('center_axis',(-4.88578146679885E-16,-1.,9.3381869947186E-16));
#43346=DIRECTION('ref_axis',(-1.,4.8857814667989E-16,5.46077161851014E-15));
#43347=DIRECTION('center_axis',(-4.88578146679885E-16,-1.,9.3381869947186E-16));
#43348=DIRECTION('ref_axis',(-1.,4.8857814667989E-16,5.46077161851014E-15));
#43349=DIRECTION('center_axis',(4.88578146679885E-16,1.,-9.3381869947186E-16));
#43350=DIRECTION('ref_axis',(-1.,4.8857814667989E-16,5.46077161851014E-15));
#43351=DIRECTION('center_axis',(-4.88578146679885E-16,-1.,9.3381869947186E-16));
#43352=DIRECTION('ref_axis',(-1.,4.8857814667989E-16,5.46077161851014E-15));
#43353=DIRECTION('center_axis',(-4.88578146679885E-16,-1.,9.3381869947186E-16));
#43354=DIRECTION('ref_axis',(-1.,4.8857814667989E-16,5.46077161851014E-15));
#43355=DIRECTION('',(-0.707106781186532,-0.707106781186563,4.60825378237839E-15));
#43356=DIRECTION('center_axis',(4.88578146679885E-16,1.,-9.3381869947186E-16));
#43357=DIRECTION('ref_axis',(1.,-4.8857814667989E-16,-5.46077161851014E-15));
#43358=DIRECTION('center_axis',(4.88578146679885E-16,1.,-9.3381869947186E-16));
#43359=DIRECTION('ref_axis',(5.46077161851014E-15,9.33818699471857E-16,
1.));
#43360=DIRECTION('',(-4.88578146679885E-16,-1.,9.3381869947186E-16));
#43361=DIRECTION('center_axis',(4.88578146679885E-16,1.,-9.3381869947186E-16));
#43362=DIRECTION('ref_axis',(5.46077161851014E-15,9.33818699471857E-16,
1.));
#43363=DIRECTION('center_axis',(-4.88578146679885E-16,-1.,9.3381869947186E-16));
#43364=DIRECTION('ref_axis',(-1.,4.8857814667989E-16,5.46077161851014E-15));
#43365=DIRECTION('center_axis',(4.88578146679885E-16,1.,-9.3381869947186E-16));
#43366=DIRECTION('ref_axis',(-1.,4.8857814667989E-16,5.46077161851014E-15));
#43367=DIRECTION('center_axis',(4.88578146679885E-16,1.,-9.3381869947186E-16));
#43368=DIRECTION('ref_axis',(-1.,4.8857814667989E-16,5.46077161851014E-15));
#43369=DIRECTION('',(-0.707106781186548,0.707106781186547,3.11444350154066E-15));
#43370=DIRECTION('center_axis',(4.88578146679885E-16,1.,-9.3381869947186E-16));
#43371=DIRECTION('ref_axis',(1.,-4.8857814667989E-16,-5.46077161851014E-15));
#43372=DIRECTION('',(-4.88578146679885E-16,-1.,9.3381869947186E-16));
#43373=DIRECTION('center_axis',(4.88578146679885E-16,1.,-9.3381869947186E-16));
#43374=DIRECTION('ref_axis',(5.46077161851014E-15,9.33818699471857E-16,
1.));
#43375=DIRECTION('center_axis',(4.88578146679885E-16,1.,-9.3381869947186E-16));
#43376=DIRECTION('ref_axis',(5.46077161851014E-15,9.33818699471857E-16,
1.));
#43377=DIRECTION('center_axis',(4.88578146679885E-16,1.,-9.3381869947186E-16));
#43378=DIRECTION('ref_axis',(-1.,4.8857814667989E-16,5.46077161851014E-15));
#43379=DIRECTION('',(-0.707106781186543,-0.707106781186552,4.60825378237844E-15));
#43380=DIRECTION('center_axis',(4.88578146679885E-16,1.,-9.3381869947186E-16));
#43381=DIRECTION('ref_axis',(-1.,4.8857814667989E-16,5.46077161851014E-15));
#43382=DIRECTION('center_axis',(-4.88578146679885E-16,-1.,9.3381869947186E-16));
#43383=DIRECTION('ref_axis',(-5.46077161851014E-15,-9.33818699471857E-16,
-1.));
#43384=DIRECTION('center_axis',(-1.,4.8857814667989E-16,5.46077161851014E-15));
#43385=DIRECTION('ref_axis',(5.46077161851014E-15,9.33818699471857E-16,
1.));
#43386=DIRECTION('',(-1.,4.8857814667989E-16,5.46077161851014E-15));
#43387=DIRECTION('center_axis',(-1.,4.8857814667989E-16,5.46077161851014E-15));
#43388=DIRECTION('ref_axis',(5.46077161851014E-15,9.33818699471857E-16,
1.));
#43389=DIRECTION('',(-1.,4.8857814667989E-16,5.46077161851014E-15));
#43390=DIRECTION('center_axis',(5.46077161851014E-15,9.33818699471857E-16,
1.));
#43391=DIRECTION('ref_axis',(4.88578146679885E-16,1.,-9.3381869947186E-16));
#43392=DIRECTION('',(4.88578146679885E-16,1.,-9.3381869947186E-16));
#43393=DIRECTION('',(4.88578146679885E-16,1.,-9.3381869947186E-16));
#43394=DIRECTION('',(-1.,4.8857814667989E-16,5.46077161851014E-15));
#43395=DIRECTION('center_axis',(-5.46077161851014E-15,-9.33818699471857E-16,
-1.));
#43396=DIRECTION('ref_axis',(-4.88578146679885E-16,-1.,9.3381869947186E-16));
#43397=DIRECTION('',(-1.,4.8857814667989E-16,5.46077161851014E-15));
#43398=DIRECTION('',(-4.88578146679885E-16,-1.,9.3381869947186E-16));
#43399=DIRECTION('center_axis',(-1.,4.8857814667989E-16,5.46077161851014E-15));
#43400=DIRECTION('ref_axis',(-5.46077161851014E-15,-9.33818699471857E-16,
-1.));
#43401=DIRECTION('center_axis',(-1.,4.8857814667989E-16,5.46077161851014E-15));
#43402=DIRECTION('ref_axis',(-5.46077161851014E-15,-9.33818699471857E-16,
-1.));
#43403=DIRECTION('center_axis',(1.,-4.8857814667989E-16,-5.46077161851014E-15));
#43404=DIRECTION('ref_axis',(-5.46077161851014E-15,-9.33818699471857E-16,
-1.));
#43405=DIRECTION('center_axis',(4.88578146679885E-16,1.,-9.3381869947186E-16));
#43406=DIRECTION('ref_axis',(1.,-4.8857814667989E-16,-5.46077161851014E-15));
#43407=DIRECTION('center_axis',(4.88578146679885E-16,1.,-9.3381869947186E-16));
#43408=DIRECTION('ref_axis',(5.46077161851014E-15,9.33818699471857E-16,
1.));
#43409=DIRECTION('center_axis',(4.88578146679885E-16,1.,-9.3381869947186E-16));
#43410=DIRECTION('ref_axis',(5.46077161851014E-15,9.33818699471857E-16,
1.));
#43411=DIRECTION('center_axis',(-4.88578146679885E-16,-1.,9.3381869947186E-16));
#43412=DIRECTION('ref_axis',(1.,-4.8857814667989E-16,-5.46077161851014E-15));
#43413=DIRECTION('',(0.707106781186543,0.707106781186552,-4.43506257113134E-15));
#43414=DIRECTION('center_axis',(4.88578146679885E-16,1.,-9.3381869947186E-16));
#43415=DIRECTION('ref_axis',(5.46077161851014E-15,9.33818699471857E-16,
1.));
#43416=DIRECTION('center_axis',(4.88578146679885E-16,1.,-9.3381869947186E-16));
#43417=DIRECTION('ref_axis',(5.46077161851014E-15,9.33818699471857E-16,
1.));
#43418=DIRECTION('center_axis',(4.88578146679885E-16,1.,-9.3381869947186E-16));
#43419=DIRECTION('ref_axis',(5.83009424213414E-15,1.45752356053353E-15,
1.));
#43420=DIRECTION('center_axis',(4.88578146679885E-16,1.,-9.3381869947186E-16));
#43421=DIRECTION('ref_axis',(5.46077161851014E-15,9.33818699471858E-16,
1.));
#43422=DIRECTION('center_axis',(1.,-4.8857814667989E-16,-5.46571335200076E-15));
#43423=DIRECTION('ref_axis',(-5.46571335200076E-15,-1.82190445066692E-15,
-1.));
#43424=DIRECTION('center_axis',(-4.88578146679885E-16,-1.,9.3381869947186E-16));
#43425=DIRECTION('ref_axis',(-5.46077161851014E-15,-9.33818699471857E-16,
-1.));
#43426=DIRECTION('center_axis',(4.88578146679885E-16,1.,-9.3381869947186E-16));
#43427=DIRECTION('ref_axis',(5.46077161851014E-15,9.33818699471857E-16,
1.));
#43428=DIRECTION('center_axis',(4.88578146679885E-16,1.,-9.3381869947186E-16));
#43429=DIRECTION('ref_axis',(1.,-4.8857814667989E-16,-5.46077161851014E-15));
#43430=DIRECTION('',(0.707106781186548,-0.707106781186547,-3.28763471278776E-15));
#43431=DIRECTION('center_axis',(-4.88578146679885E-16,-1.,9.3381869947186E-16));
#43432=DIRECTION('ref_axis',(1.,-4.8857814667989E-16,-5.46077161851014E-15));
#43433=DIRECTION('',(0.707106781186549,0.707106781186546,-4.43506257113137E-15));
#43434=DIRECTION('center_axis',(4.88578146679885E-16,1.,-9.3381869947186E-16));
#43435=DIRECTION('ref_axis',(5.46077161851014E-15,9.33818699471857E-16,
1.));
#43436=DIRECTION('center_axis',(4.88578146679885E-16,1.,-9.3381869947186E-16));
#43437=DIRECTION('ref_axis',(5.46077161851014E-15,9.33818699471857E-16,
1.));
#43438=DIRECTION('center_axis',(4.88578146679885E-16,1.,-9.3381869947186E-16));
#43439=DIRECTION('ref_axis',(5.46077161851014E-15,9.33818699471858E-16,
1.));
#43440=DIRECTION('center_axis',(4.88578146679885E-16,1.,-9.3381869947186E-16));
#43441=DIRECTION('ref_axis',(5.83009424213416E-15,7.28761780266769E-16,
1.));
#43442=DIRECTION('center_axis',(1.,-4.8857814667989E-16,-5.46571335200076E-15));
#43443=DIRECTION('ref_axis',(-5.46571335200076E-15,-9.10952225333461E-16,
-1.));
#55888=CARTESIAN_POINT('',(0.,0.,0.));
#55889=CARTESIAN_POINT('Origin',(263.115917770968,-180.47200726879,445.000000551893));
#55890=CARTESIAN_POINT('',(243.115917770968,-105.97200726879,445.000000551893));
#55891=CARTESIAN_POINT('',(243.115917770968,-254.97200726879,445.000000551893));
#55892=CARTESIAN_POINT('',(243.115917770968,-180.47200726879,445.000000551893));
#55893=CARTESIAN_POINT('',(283.115917770968,-105.97200726879,445.000000551893));
#55894=CARTESIAN_POINT('Origin',(263.115917770968,-105.97200726879,445.000000551893));
#55895=CARTESIAN_POINT('',(282.194701799307,-111.97200726879,439.000000551893));
#55896=CARTESIAN_POINT('Ctrl Pts',(283.115917770968,-105.97200726879,445.000000551893));
#55897=CARTESIAN_POINT('Ctrl Pts',(283.115917770968,-105.97200726879,444.241672021309));
#55898=CARTESIAN_POINT('Ctrl Pts',(283.068520438725,-106.124510775769,443.435925116929));
#55899=CARTESIAN_POINT('Ctrl Pts',(282.89734167077,-106.738309454724,441.958955713881));
#55900=CARTESIAN_POINT('Ctrl Pts',(282.775789023268,-107.199354583986,441.287371862459));
#55901=CARTESIAN_POINT('Ctrl Pts',(282.545652805548,-108.259536519781,440.227189926664));
#55902=CARTESIAN_POINT('Ctrl Pts',(282.421616893032,-108.931056193358,439.766267099578));
#55903=CARTESIAN_POINT('Ctrl Pts',(282.244676552118,-110.407792297934,439.152558719695));
#55904=CARTESIAN_POINT('Ctrl Pts',(282.194701799307,-111.213452760811,439.000000551893));
#55905=CARTESIAN_POINT('Ctrl Pts',(282.194701799307,-111.97200726879,439.000000551893));
#55906=CARTESIAN_POINT('',(282.194701799307,-248.97200726879,439.000000551893));
#55907=CARTESIAN_POINT('',(282.194701799307,-180.47200726879,439.000000551893));
#55908=CARTESIAN_POINT('',(283.115917770968,-254.97200726879,445.000000551893));
#55909=CARTESIAN_POINT('Ctrl Pts',(282.194701799307,-248.97200726879,439.000000551893));
#55910=CARTESIAN_POINT('Ctrl Pts',(282.194701799307,-249.730561776769,439.000000551893));
#55911=CARTESIAN_POINT('Ctrl Pts',(282.244676552118,-250.536222239646,439.152558719695));
#55912=CARTESIAN_POINT('Ctrl Pts',(282.421616893032,-252.012958344222,439.766267099578));
#55913=CARTESIAN_POINT('Ctrl Pts',(282.545652805548,-252.684478017799,440.227189926664));
#55914=CARTESIAN_POINT('Ctrl Pts',(282.775789023268,-253.744659953594,441.287371862459));
#55915=CARTESIAN_POINT('Ctrl Pts',(282.89734167077,-254.205705082856,441.958955713881));
#55916=CARTESIAN_POINT('Ctrl Pts',(283.068520438725,-254.819503761811,443.435925116929));
#55917=CARTESIAN_POINT('Ctrl Pts',(283.115917770968,-254.97200726879,444.241672021309));
#55918=CARTESIAN_POINT('Ctrl Pts',(283.115917770968,-254.97200726879,445.000000551893));
#55919=CARTESIAN_POINT('Origin',(263.115917770968,-254.97200726879,445.000000551893));
#55920=CARTESIAN_POINT('Origin',(278.115917770968,9.52799273120991,445.000000551893));
#55921=CARTESIAN_POINT('',(276.863644855836,9.52799273120991,451.000000551893));
#55922=CARTESIAN_POINT('',(276.863644855836,9.52799273120991,439.000000551893));
#55923=CARTESIAN_POINT('Ctrl Pts',(276.863644855836,9.52799273120992,451.000000551893));
#55924=CARTESIAN_POINT('Ctrl Pts',(276.863644855836,10.2911080617152,451.000000551893));
#55925=CARTESIAN_POINT('Ctrl Pts',(276.933905272325,11.0983145255455,450.845735154055));
#55926=CARTESIAN_POINT('Ctrl Pts',(277.178138317006,12.5735133048384,450.230998285314));
#55927=CARTESIAN_POINT('Ctrl Pts',(277.347642076354,13.2423907504513,449.77088390689));
#55928=CARTESIAN_POINT('Ctrl Pts',(277.659025023679,14.2983417003919,448.714932956949));
#55929=CARTESIAN_POINT('Ctrl Pts',(277.822400067743,14.7588613493959,448.045853243948));
#55930=CARTESIAN_POINT('Ctrl Pts',(278.05222803659,15.3739084341755,446.569865474975));
#55931=CARTESIAN_POINT('Ctrl Pts',(278.115917770968,15.5279927312099,445.762343892491));
#55932=CARTESIAN_POINT('Ctrl Pts',(278.115917770968,15.5279927312099,444.237657211294));
#55933=CARTESIAN_POINT('Ctrl Pts',(278.05222803659,15.3739084341755,443.430135628811));
#55934=CARTESIAN_POINT('Ctrl Pts',(277.822400067743,14.7588613493959,441.954147859838));
#55935=CARTESIAN_POINT('Ctrl Pts',(277.659025023679,14.2983417003919,441.285068146836));
#55936=CARTESIAN_POINT('Ctrl Pts',(277.347642076353,13.2423907504513,440.229117196896));
#55937=CARTESIAN_POINT('Ctrl Pts',(277.178138317006,12.5735133048384,439.769002818472));
#55938=CARTESIAN_POINT('Ctrl Pts',(276.933905272324,11.0983145255455,439.154265949731));
#55939=CARTESIAN_POINT('Ctrl Pts',(276.863644855836,10.2911080617152,439.000000551893));
#55940=CARTESIAN_POINT('Ctrl Pts',(276.863644855836,9.52799273120991,439.000000551893));
#55941=CARTESIAN_POINT('',(270.115917770968,9.52799273120991,451.000000551893));
#55942=CARTESIAN_POINT('',(278.115917770968,9.52799273120991,451.000000551893));
#55943=CARTESIAN_POINT('',(270.115917770968,9.52799273120991,439.000000551893));
#55944=CARTESIAN_POINT('Origin',(270.115917770968,9.52799273120991,445.000000551893));
#55945=CARTESIAN_POINT('',(278.115917770968,9.52799273120991,439.000000551893));
#55946=CARTESIAN_POINT('Origin',(278.115917770968,9.52799273120991,439.000000551893));
#55947=CARTESIAN_POINT('',(276.863644855836,-20.4720072687901,439.000000551893));
#55948=CARTESIAN_POINT('',(276.863644855836,-39.9720072687901,439.000000551893));
#55949=CARTESIAN_POINT('',(270.115917770968,-20.4720072687901,439.000000551893));
#55950=CARTESIAN_POINT('',(270.115917770968,-20.4720072687901,439.000000551893));
#55951=CARTESIAN_POINT('',(278.115917770968,-20.4720072687901,439.000000551893));
#55952=CARTESIAN_POINT('Origin',(278.115917770968,-20.4720072687901,451.000000551893));
#55953=CARTESIAN_POINT('',(276.863644855836,-20.4720072687901,451.000000551893));
#55954=CARTESIAN_POINT('',(276.863644855836,-39.9720072687901,451.000000551893));
#55955=CARTESIAN_POINT('',(270.115917770968,-20.4720072687901,451.000000551893));
#55956=CARTESIAN_POINT('',(278.115917770968,-20.4720072687901,451.000000551893));
#55957=CARTESIAN_POINT('',(270.115917770968,9.52799273120991,451.000000551893));
#55958=CARTESIAN_POINT('Origin',(278.115917770968,-20.4720072687901,445.000000551893));
#55959=CARTESIAN_POINT('Ctrl Pts',(276.863644855836,-20.4720072687901,451.000000551893));
#55960=CARTESIAN_POINT('Ctrl Pts',(276.863644855836,-21.2351225992954,451.000000551893));
#55961=CARTESIAN_POINT('Ctrl Pts',(276.933905272325,-22.0423290631257,450.845735154055));
#55962=CARTESIAN_POINT('Ctrl Pts',(277.178138317006,-23.5175278424185,450.230998285314));
#55963=CARTESIAN_POINT('Ctrl Pts',(277.347642076354,-24.1864052880315,449.77088390689));
#55964=CARTESIAN_POINT('Ctrl Pts',(277.659025023679,-25.2423562379721,448.71493295695));
#55965=CARTESIAN_POINT('Ctrl Pts',(277.822400067743,-25.702875886976,448.045853243948));
#55966=CARTESIAN_POINT('Ctrl Pts',(278.05222803659,-26.3179229717557,446.569865474975));
#55967=CARTESIAN_POINT('Ctrl Pts',(278.115917770968,-26.4720072687901,445.762343892492));
#55968=CARTESIAN_POINT('Ctrl Pts',(278.115917770968,-26.4720072687901,444.237657211294));
#55969=CARTESIAN_POINT('Ctrl Pts',(278.05222803659,-26.3179229717557,443.430135628811));
#55970=CARTESIAN_POINT('Ctrl Pts',(277.822400067743,-25.702875886976,441.954147859838));
#55971=CARTESIAN_POINT('Ctrl Pts',(277.659025023679,-25.2423562379721,441.285068146836));
#55972=CARTESIAN_POINT('Ctrl Pts',(277.347642076353,-24.1864052880315,440.229117196896));
#55973=CARTESIAN_POINT('Ctrl Pts',(277.178138317006,-23.5175278424185,439.769002818472));
#55974=CARTESIAN_POINT('Ctrl Pts',(276.933905272324,-22.0423290631256,439.154265949731));
#55975=CARTESIAN_POINT('Ctrl Pts',(276.863644855836,-21.2351225992954,439.000000551893));
#55976=CARTESIAN_POINT('Ctrl Pts',(276.863644855836,-20.4720072687901,439.000000551893));
#55977=CARTESIAN_POINT('Origin',(270.115917770968,-20.4720072687901,445.000000551893));
#55978=CARTESIAN_POINT('Origin',(270.115917770968,-5.47200726879009,445.000000551893));
#55979=CARTESIAN_POINT('Origin',(263.115917770968,-98.97200726879,445.000000551893));
#55980=CARTESIAN_POINT('',(263.115917770968,-98.97200726879,430.000000551893));
#55981=CARTESIAN_POINT('',(248.115917770968,-98.97200726879,445.000000551893));
#55982=CARTESIAN_POINT('Origin',(263.115917770968,-98.97200726879,445.000000551893));
#55983=CARTESIAN_POINT('Origin',(263.115917770968,-98.97200726879,445.000000551893));
#55984=CARTESIAN_POINT('',(263.115917770968,-99.47200726879,429.500000551893));
#55985=CARTESIAN_POINT('Origin',(263.115917770968,-98.97200726879,429.500000551893));
#55986=CARTESIAN_POINT('Origin',(263.115917770968,-99.47200726879,445.000000551893));
#55987=CARTESIAN_POINT('Origin',(278.115917770968,-99.47200726879,445.000000551893));
#55988=CARTESIAN_POINT('',(281.115917770968,-99.47200726879,445.000000551893));
#55989=CARTESIAN_POINT('Origin',(263.115917770968,-99.47200726879,445.000000551893));
#55990=CARTESIAN_POINT('Origin',(263.115917770968,-39.9720072687901,445.000000551893));
#55991=CARTESIAN_POINT('',(248.115917770968,19.52799273121,445.000000551893));
#55992=CARTESIAN_POINT('Origin',(263.115917770968,19.5279927312099,445.000000551893));
#55993=CARTESIAN_POINT('',(248.115917770968,-39.9720072687901,445.000000551893));
#55994=CARTESIAN_POINT('Origin',(263.115917770968,-261.47200726879,445.000000551893));
#55995=CARTESIAN_POINT('',(263.115917770968,-260.97200726879,429.500000551893));
#55996=CARTESIAN_POINT('Origin',(263.115917770968,-260.97200726879,445.000000551893));
#55997=CARTESIAN_POINT('',(263.115917770968,-261.47200726879,430.000000551893));
#55998=CARTESIAN_POINT('Origin',(263.115917770968,-261.47200726879,429.500000551893));
#55999=CARTESIAN_POINT('',(248.115917770968,-261.47200726879,445.000000551893));
#56000=CARTESIAN_POINT('Origin',(263.115917770968,-261.47200726879,445.000000551893));
#56001=CARTESIAN_POINT('Origin',(263.115917770968,-261.47200726879,445.000000551893));
#56002=CARTESIAN_POINT('Origin',(281.615917770968,-260.97200726879,445.000000551893));
#56003=CARTESIAN_POINT('',(281.115917770968,-260.97200726879,445.000000551893));
#56004=CARTESIAN_POINT('Origin',(263.115917770968,-260.97200726879,445.000000551893));
#56005=CARTESIAN_POINT('Origin',(263.115917770968,-295.97200726879,445.000000551893));
#56006=CARTESIAN_POINT('',(248.115917770968,-329.97200726879,445.000000551893));
#56007=CARTESIAN_POINT('',(248.115917770968,-295.97200726879,445.000000551893));
#56008=CARTESIAN_POINT('',(278.115917770968,-329.97200726879,445.000000551893));
#56009=CARTESIAN_POINT('Origin',(263.115917770968,-329.97200726879,445.000000551893));
#56010=CARTESIAN_POINT('Origin',(263.115917770968,-329.97200726879,445.000000551893));
#56011=CARTESIAN_POINT('Origin',(263.115917770968,-260.72200726879,445.000000551893));
#56012=CARTESIAN_POINT('',(281.615917770968,-260.47200726879,445.000000551893));
#56013=CARTESIAN_POINT('',(244.615917770968,-260.47200726879,445.000000551893));
#56014=CARTESIAN_POINT('Origin',(263.115917770968,-260.47200726879,445.000000551893));
#56015=CARTESIAN_POINT('Origin',(263.115917770968,-260.47200726879,445.000000551893));
#56016=CARTESIAN_POINT('',(281.365917770968,-260.72200726879,445.000000551893));
#56017=CARTESIAN_POINT('Origin',(263.115917770968,-258.47200726879,445.000000551893));
#56018=CARTESIAN_POINT('',(244.615917770968,-255.97200726879,445.000000551893));
#56019=CARTESIAN_POINT('',(263.115917770968,-255.97200726879,426.500000551893));
#56020=CARTESIAN_POINT('Origin',(263.115917770968,-255.97200726879,445.000000551893));
#56021=CARTESIAN_POINT('',(244.615917770968,-258.47200726879,445.000000551893));
#56022=CARTESIAN_POINT('Origin',(263.115917770968,-255.97200726879,445.000000551893));
#56023=CARTESIAN_POINT('Origin',(263.115917770968,-99.72200726879,445.000000551893));
#56024=CARTESIAN_POINT('',(281.615917770968,-99.97200726879,445.000000551893));
#56025=CARTESIAN_POINT('',(244.615917770968,-99.97200726879,445.000000551893));
#56026=CARTESIAN_POINT('Origin',(263.115917770968,-99.97200726879,445.000000551893));
#56027=CARTESIAN_POINT('Origin',(263.115917770968,-99.97200726879,445.000000551893));
#56028=CARTESIAN_POINT('',(281.365917770968,-99.72200726879,445.000000551893));
#56029=CARTESIAN_POINT('Origin',(263.115917770968,-102.22200726879,445.000000551893));
#56030=CARTESIAN_POINT('',(244.615917770968,-104.97200726879,445.000000551893));
#56031=CARTESIAN_POINT('',(244.615917770968,-102.22200726879,445.000000551893));
#56032=CARTESIAN_POINT('',(263.115917770968,-104.97200726879,426.500000551893));
#56033=CARTESIAN_POINT('Origin',(263.115917770968,-104.97200726879,445.000000551893));
#56034=CARTESIAN_POINT('Origin',(263.115917770968,-104.97200726879,445.000000551893));
#56035=CARTESIAN_POINT('Origin',(263.115917770968,-330.47200726879,445.000000551893));
#56036=CARTESIAN_POINT('',(277.115917770968,-330.97200726879,445.000000551893));
#56037=CARTESIAN_POINT('',(277.615917770968,-330.47200726879,445.000000551893));
#56038=CARTESIAN_POINT('Origin',(263.115917770968,-330.97200726879,445.000000551893));
#56039=CARTESIAN_POINT('Origin',(278.115917770968,-330.97200726879,445.000000551893));
#56040=CARTESIAN_POINT('Origin',(283.115917770968,-248.97200726879,445.000000551893));
#56041=CARTESIAN_POINT('',(275.115917770968,-248.97200726879,439.000000551893));
#56042=CARTESIAN_POINT('',(283.115917770968,-248.97200726879,439.000000551893));
#56043=CARTESIAN_POINT('',(275.115917770968,-248.97200726879,451.000000551893));
#56044=CARTESIAN_POINT('Origin',(275.115917770968,-248.97200726879,445.000000551893));
#56045=CARTESIAN_POINT('',(282.194701799307,-248.97200726879,451.000000551893));
#56046=CARTESIAN_POINT('',(283.115917770968,-248.97200726879,451.000000551893));
#56047=CARTESIAN_POINT('Ctrl Pts',(283.115917770968,-254.97200726879,445.000000551893));
#56048=CARTESIAN_POINT('Ctrl Pts',(283.115917770968,-254.97200726879,445.758329082477));
#56049=CARTESIAN_POINT('Ctrl Pts',(283.068520438725,-254.819503761811,446.564075986857));
#56050=CARTESIAN_POINT('Ctrl Pts',(282.89734167077,-254.205705082856,448.041045389906));
#56051=CARTESIAN_POINT('Ctrl Pts',(282.775789023268,-253.744659953594,448.712629241327));
#56052=CARTESIAN_POINT('Ctrl Pts',(282.545652805548,-252.684478017799,449.772811177122));
#56053=CARTESIAN_POINT('Ctrl Pts',(282.421616893032,-252.012958344222,450.233734004208));
#56054=CARTESIAN_POINT('Ctrl Pts',(282.244676552118,-250.536222239646,450.847442384092));
#56055=CARTESIAN_POINT('Ctrl Pts',(282.194701799307,-249.730561776768,451.000000551893));
#56056=CARTESIAN_POINT('Ctrl Pts',(282.194701799307,-248.97200726879,451.000000551893));
#56057=CARTESIAN_POINT('Origin',(283.115917770968,-248.97200726879,451.000000551893));
#56058=CARTESIAN_POINT('',(282.194701799307,-111.97200726879,451.000000551893));
#56059=CARTESIAN_POINT('',(282.194701799307,-180.47200726879,451.000000551893));
#56060=CARTESIAN_POINT('',(275.115917770968,-111.97200726879,451.000000551893));
#56061=CARTESIAN_POINT('',(275.115917770968,-111.97200726879,451.000000551893));
#56062=CARTESIAN_POINT('',(283.115917770968,-111.97200726879,451.000000551893));
#56063=CARTESIAN_POINT('Origin',(283.115917770968,-111.97200726879,439.000000551893));
#56064=CARTESIAN_POINT('',(275.115917770968,-111.97200726879,439.000000551893));
#56065=CARTESIAN_POINT('',(283.115917770968,-111.97200726879,439.000000551893));
#56066=CARTESIAN_POINT('',(275.115917770968,-248.97200726879,439.000000551893));
#56067=CARTESIAN_POINT('Origin',(283.115917770968,-111.97200726879,445.000000551893));
#56068=CARTESIAN_POINT('Ctrl Pts',(282.194701799307,-111.97200726879,451.000000551893));
#56069=CARTESIAN_POINT('Ctrl Pts',(282.194701799307,-111.213452760811,451.000000551893));
#56070=CARTESIAN_POINT('Ctrl Pts',(282.244676552118,-110.407792297934,450.847442384091));
#56071=CARTESIAN_POINT('Ctrl Pts',(282.421616893032,-108.931056193358,450.233734004208));
#56072=CARTESIAN_POINT('Ctrl Pts',(282.545652805548,-108.259536519781,449.772811177122));
#56073=CARTESIAN_POINT('Ctrl Pts',(282.775789023268,-107.199354583986,448.712629241327));
#56074=CARTESIAN_POINT('Ctrl Pts',(282.89734167077,-106.738309454724,448.041045389905));
#56075=CARTESIAN_POINT('Ctrl Pts',(283.068520438725,-106.124510775769,446.564075986857));
#56076=CARTESIAN_POINT('Ctrl Pts',(283.115917770968,-105.97200726879,445.758329082477));
#56077=CARTESIAN_POINT('Ctrl Pts',(283.115917770968,-105.97200726879,445.000000551893));
#56078=CARTESIAN_POINT('Origin',(275.115917770968,-111.97200726879,445.000000551893));
#56079=CARTESIAN_POINT('Origin',(275.115917770968,-180.47200726879,445.000000551893));
#56080=CARTESIAN_POINT('Origin',(263.115917770968,-180.47200726879,445.000000551893));
#56081=CARTESIAN_POINT('Origin',(263.115917770968,-254.97200726879,445.000000551893));
#56082=CARTESIAN_POINT('Origin',(263.115917770968,-105.97200726879,445.000000551893));
#56083=CARTESIAN_POINT('Origin',(263.115917770968,20.0279927312099,445.000000551893));
#56084=CARTESIAN_POINT('',(249.115917770968,20.52799273121,445.000000551893));
#56085=CARTESIAN_POINT('',(248.615917770968,20.0279927312099,445.000000551893));
#56086=CARTESIAN_POINT('Origin',(263.115917770968,20.5279927312099,445.000000551893));
#56087=CARTESIAN_POINT('Origin',(263.115917770968,20.5279927312099,445.000000551893));
#56088=CARTESIAN_POINT('Origin',(263.115917770968,-255.97200726879,445.000000551893));
#56089=CARTESIAN_POINT('',(263.115917770968,-255.47200726879,426.000000551893));
#56090=CARTESIAN_POINT('Origin',(263.115917770968,-255.47200726879,445.000000551893));
#56091=CARTESIAN_POINT('Origin',(263.115917770968,-255.97200726879,426.000000551893));
#56092=CARTESIAN_POINT('Origin',(282.615917770968,-255.47200726879,445.000000551893));
#56093=CARTESIAN_POINT('',(243.615917770968,-255.47200726879,445.000000551893));
#56094=CARTESIAN_POINT('Origin',(263.115917770968,-255.47200726879,445.000000551893));
#56095=CARTESIAN_POINT('Origin',(263.115917770968,-255.22200726879,445.000000551893));
#56096=CARTESIAN_POINT('',(243.365917770968,-255.22200726879,445.000000551893));
#56097=CARTESIAN_POINT('Origin',(263.115917770968,-105.72200726879,445.000000551893));
#56098=CARTESIAN_POINT('',(243.615917770968,-105.47200726879,445.000000551893));
#56099=CARTESIAN_POINT('',(243.365917770968,-105.72200726879,445.000000551893));
#56100=CARTESIAN_POINT('Origin',(263.115917770968,-105.47200726879,445.000000551893));
#56101=CARTESIAN_POINT('Origin',(282.115917770968,-105.47200726879,445.000000551893));
#56102=CARTESIAN_POINT('',(263.115917770968,-105.47200726879,426.000000551893));
#56103=CARTESIAN_POINT('Origin',(263.115917770968,-105.47200726879,445.000000551893));
#56104=CARTESIAN_POINT('Origin',(263.115917770968,-104.97200726879,445.000000551893));
#56105=CARTESIAN_POINT('Origin',(263.115917770968,-104.97200726879,426.000000551893));
#61770=UNCERTAINTY_MEASURE_WITH_UNIT(LENGTH_MEASURE(0.01),#61812,
'DISTANCE_ACCURACY_VALUE',
'Maximum model space distance between geometric entities at asserted c
onnectivities');
#61780=UNCERTAINTY_MEASURE_WITH_UNIT(LENGTH_MEASURE(0.01),#61812,
'DISTANCE_ACCURACY_VALUE',
'Maximum model space distance between geometric entities at asserted c
onnectivities');
#61801=(
GEOMETRIC_REPRESENTATION_CONTEXT(3)
GLOBAL_UNCERTAINTY_ASSIGNED_CONTEXT((#61770))
GLOBAL_UNIT_ASSIGNED_CONTEXT((#61812,#61814,#61815))
REPRESENTATION_CONTEXT('','3D')
);
#61811=(
GEOMETRIC_REPRESENTATION_CONTEXT(3)
GLOBAL_UNCERTAINTY_ASSIGNED_CONTEXT((#61780))
GLOBAL_UNIT_ASSIGNED_CONTEXT((#61812,#61814,#61815))
REPRESENTATION_CONTEXT('','3D')
);
#61812=(
LENGTH_UNIT()
NAMED_UNIT(*)
SI_UNIT(.MILLI.,.METRE.)
);
#61814=(
NAMED_UNIT(*)
PLANE_ANGLE_UNIT()
SI_UNIT($,.RADIAN.)
);
#61815=(
NAMED_UNIT(*)
SI_UNIT($,.STERADIAN.)
SOLID_ANGLE_UNIT()
);
#61836=SHAPE_DEFINITION_REPRESENTATION(#61882,#61988);
#61882=PRODUCT_DEFINITION_SHAPE('',$,#62019);
#61988=SHAPE_REPRESENTATION('',(#35962),#61801);
#61998=PRODUCT_DEFINITION_CONTEXT('part definition',#62090,'design');
#62019=PRODUCT_DEFINITION('Cutter Shaft A','Cutter Shaft A',#62049,#61998);
#62049=PRODUCT_DEFINITION_FORMATION('',$,#62112);
#62090=APPLICATION_CONTEXT('Managed model based 3d engineering');
#62091=PRODUCT_CONTEXT('part definition',#62090,'mechanical');
#62112=PRODUCT('Cutter Shaft A','Cutter Shaft A',$,(#62091));
#62150=COLOUR_RGB('Grey',0.48,0.52,0.57);
#62151=FILL_AREA_STYLE_COLOUR('',#62150);
#62152=FILL_AREA_STYLE('',(#62151));
#62153=SURFACE_STYLE_FILL_AREA(#62152);
#62154=SURFACE_SIDE_STYLE('',(#62153));
#62155=SURFACE_STYLE_USAGE(.BOTH.,#62154);
#62156=PRESENTATION_STYLE_ASSIGNMENT((#62155));
ENDSEC;
END-ISO-10303-21;
